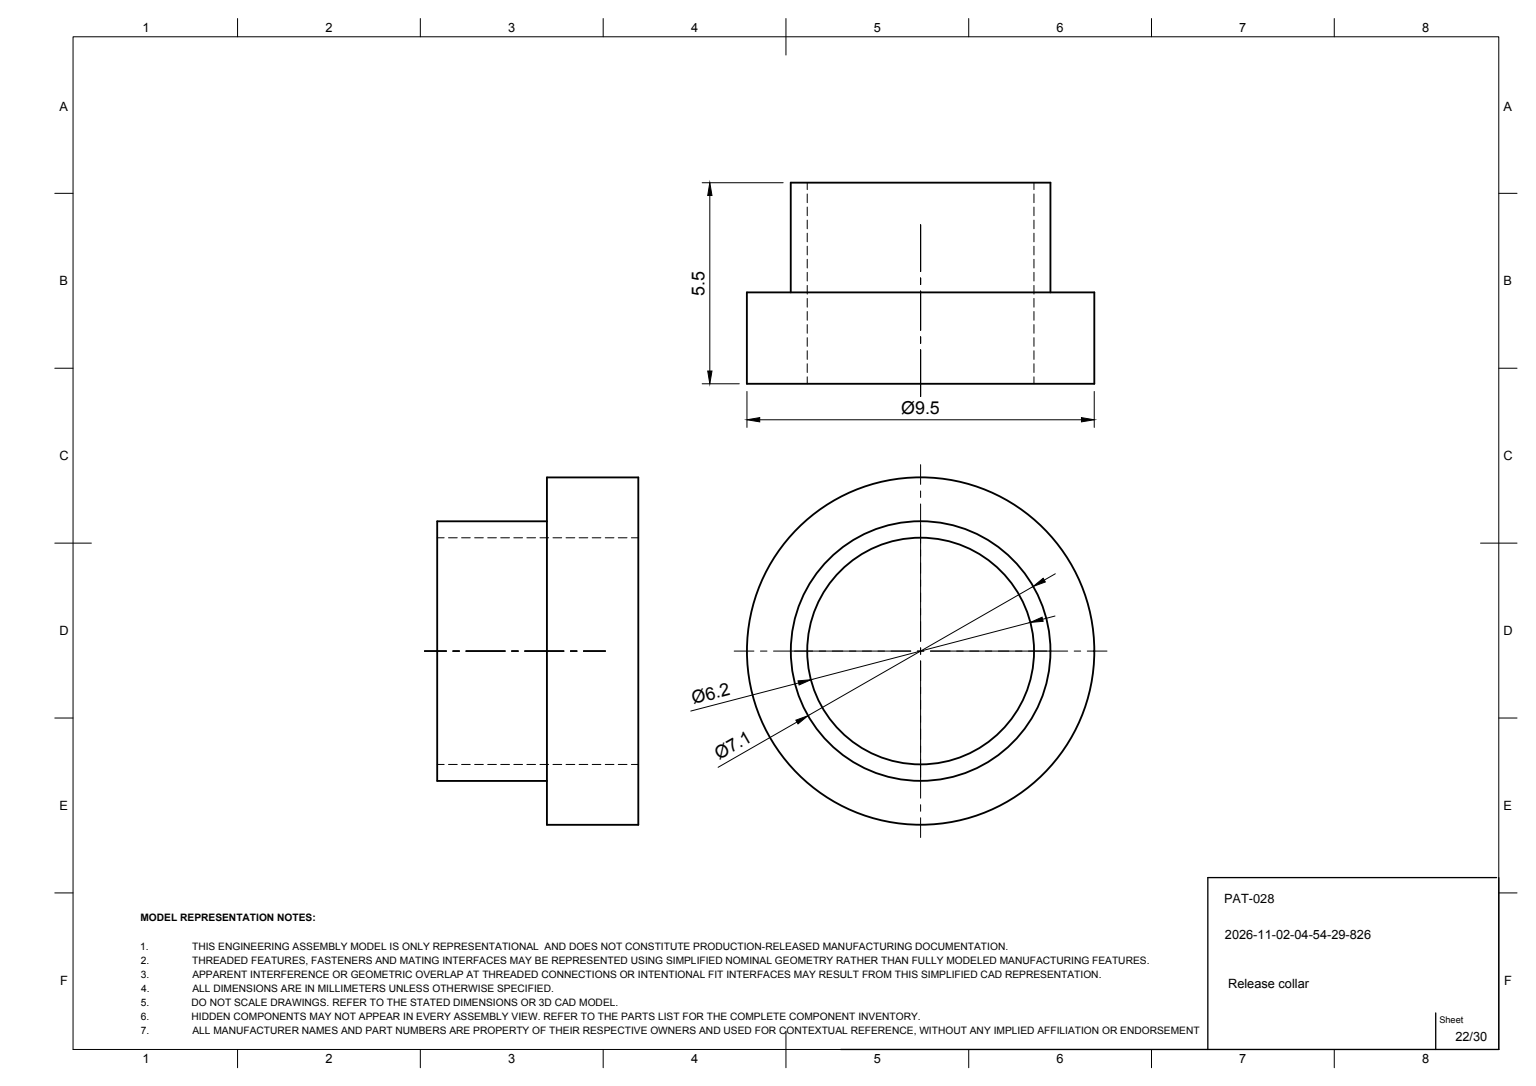
ISO-10303-21;
HEADER;
/* Generated by software containing ST-Developer
 * from STEP Tools, Inc. (www.steptools.com) 
 */

FILE_DESCRIPTION(
/* description */ ('Cylinder foot and clevis mount kit'),
/* implementation_level */ '2;1');

FILE_NAME(
/* name */ 'Release collar.step',
/* time_stamp */ '2026-10-27T20:10:43-07:00',
/* author */ (''),
/* organization */ (''),
/* preprocessor_version */ 'ST-DEVELOPER v20.2',
/* originating_system */ 'Autodesk Translation Framework v15.17.0.0',
/* authorisation */ '');

FILE_SCHEMA (('AUTOMOTIVE_DESIGN { 1 0 10303 214 3 1 1 }'));
ENDSEC;

DATA;
#10=MECHANICAL_DESIGN_GEOMETRIC_PRESENTATION_REPRESENTATION('',(#350),#9102);
#294=SHAPE_REPRESENTATION_RELATIONSHIP('SRR','None',#9242,#322);
#322=ADVANCED_BREP_SHAPE_REPRESENTATION('',(#377),#9085);
#350=STYLED_ITEM('',(#9474),#377);
#377=MANIFOLD_SOLID_BREP('Body1',#4937);
#463=FACE_BOUND('',#1266,.T.);
#464=FACE_BOUND('',#1269,.T.);
#465=FACE_BOUND('',#1272,.T.);
#628=PLANE('',#5624);
#629=PLANE('',#5629);
#630=PLANE('',#5633);
#888=FACE_OUTER_BOUND('',#1265,.T.);
#889=FACE_OUTER_BOUND('',#1267,.T.);
#890=FACE_OUTER_BOUND('',#1268,.T.);
#891=FACE_OUTER_BOUND('',#1270,.T.);
#892=FACE_OUTER_BOUND('',#1271,.T.);
#893=FACE_OUTER_BOUND('',#1273,.T.);
#1265=EDGE_LOOP('',(#4087));
#1266=EDGE_LOOP('',(#4088));
#1267=EDGE_LOOP('',(#4089,#4090,#4091,#4092));
#1268=EDGE_LOOP('',(#4093));
#1269=EDGE_LOOP('',(#4094));
#1270=EDGE_LOOP('',(#4095,#4096,#4097,#4098));
#1271=EDGE_LOOP('',(#4099));
#1272=EDGE_LOOP('',(#4100));
#1273=EDGE_LOOP('',(#4101,#4102,#4103,#4104));
#1644=LINE('',#8343,#1993);
#1645=LINE('',#8350,#1994);
#1646=LINE('',#8355,#1995);
#1993=VECTOR('',#6857,0.475);
#1994=VECTOR('',#6866,0.355);
#1995=VECTOR('',#6873,0.31);
#2246=CIRCLE('',#5625,0.475);
#2247=CIRCLE('',#5626,0.31);
#2248=CIRCLE('',#5628,0.475);
#2249=CIRCLE('',#5630,0.355);
#2250=CIRCLE('',#5632,0.355);
#2251=CIRCLE('',#5634,0.31);
#2572=VERTEX_POINT('',#8336);
#2573=VERTEX_POINT('',#8338);
#2574=VERTEX_POINT('',#8341);
#2575=VERTEX_POINT('',#8345);
#2576=VERTEX_POINT('',#8348);
#2577=VERTEX_POINT('',#8352);
#3098=EDGE_CURVE('',#2572,#2572,#2246,.T.);
#3099=EDGE_CURVE('',#2573,#2573,#2247,.T.);
#3100=EDGE_CURVE('',#2574,#2574,#2248,.T.);
#3101=EDGE_CURVE('',#2574,#2572,#1644,.T.);
#3102=EDGE_CURVE('',#2575,#2575,#2249,.T.);
#3103=EDGE_CURVE('',#2576,#2576,#2250,.T.);
#3104=EDGE_CURVE('',#2576,#2575,#1645,.T.);
#3105=EDGE_CURVE('',#2577,#2577,#2251,.T.);
#3106=EDGE_CURVE('',#2577,#2573,#1646,.T.);
#4087=ORIENTED_EDGE('',*,*,#3098,.F.);
#4088=ORIENTED_EDGE('',*,*,#3099,.T.);
#4089=ORIENTED_EDGE('',*,*,#3100,.F.);
#4090=ORIENTED_EDGE('',*,*,#3101,.T.);
#4091=ORIENTED_EDGE('',*,*,#3098,.T.);
#4092=ORIENTED_EDGE('',*,*,#3101,.F.);
#4093=ORIENTED_EDGE('',*,*,#3100,.T.);
#4094=ORIENTED_EDGE('',*,*,#3102,.F.);
#4095=ORIENTED_EDGE('',*,*,#3103,.F.);
#4096=ORIENTED_EDGE('',*,*,#3104,.T.);
#4097=ORIENTED_EDGE('',*,*,#3102,.T.);
#4098=ORIENTED_EDGE('',*,*,#3104,.F.);
#4099=ORIENTED_EDGE('',*,*,#3103,.T.);
#4100=ORIENTED_EDGE('',*,*,#3105,.F.);
#4101=ORIENTED_EDGE('',*,*,#3105,.T.);
#4102=ORIENTED_EDGE('',*,*,#3106,.T.);
#4103=ORIENTED_EDGE('',*,*,#3099,.F.);
#4104=ORIENTED_EDGE('',*,*,#3106,.F.);
#4587=CYLINDRICAL_SURFACE('',#5627,0.475);
#4588=CYLINDRICAL_SURFACE('',#5631,0.355);
#4589=CYLINDRICAL_SURFACE('',#5635,0.31);
#4811=ADVANCED_FACE('',(#888,#463),#628,.T.);
#4812=ADVANCED_FACE('',(#889),#4587,.T.);
#4813=ADVANCED_FACE('',(#890,#464),#629,.T.);
#4814=ADVANCED_FACE('',(#891),#4588,.T.);
#4815=ADVANCED_FACE('',(#892,#465),#630,.T.);
#4816=ADVANCED_FACE('',(#893),#4589,.F.);
#4937=CLOSED_SHELL('',(#4811,#4812,#4813,#4814,#4815,#4816));
#5623=AXIS2_PLACEMENT_3D('',#8334,#6845,#6846);
#5624=AXIS2_PLACEMENT_3D('',#8335,#6847,#6848);
#5625=AXIS2_PLACEMENT_3D('',#8337,#6849,#6850);
#5626=AXIS2_PLACEMENT_3D('',#8339,#6851,#6852);
#5627=AXIS2_PLACEMENT_3D('',#8340,#6853,#6854);
#5628=AXIS2_PLACEMENT_3D('',#8342,#6855,#6856);
#5629=AXIS2_PLACEMENT_3D('',#8344,#6858,#6859);
#5630=AXIS2_PLACEMENT_3D('',#8346,#6860,#6861);
#5631=AXIS2_PLACEMENT_3D('',#8347,#6862,#6863);
#5632=AXIS2_PLACEMENT_3D('',#8349,#6864,#6865);
#5633=AXIS2_PLACEMENT_3D('',#8351,#6867,#6868);
#5634=AXIS2_PLACEMENT_3D('',#8353,#6869,#6870);
#5635=AXIS2_PLACEMENT_3D('',#8354,#6871,#6872);
#6845=DIRECTION('axis',(0.,0.,1.));
#6846=DIRECTION('refdir',(1.,0.,0.));
#6847=DIRECTION('center_axis',(0.,1.,0.));
#6848=DIRECTION('ref_axis',(0.,0.,1.));
#6849=DIRECTION('center_axis',(0.,-1.,0.));
#6850=DIRECTION('ref_axis',(1.,0.,0.));
#6851=DIRECTION('center_axis',(0.,-1.,0.));
#6852=DIRECTION('ref_axis',(1.,0.,0.));
#6853=DIRECTION('center_axis',(0.,-1.,0.));
#6854=DIRECTION('ref_axis',(1.,0.,0.));
#6855=DIRECTION('center_axis',(0.,-1.,0.));
#6856=DIRECTION('ref_axis',(1.,0.,0.));
#6857=DIRECTION('',(0.,1.,0.));
#6858=DIRECTION('center_axis',(0.,-1.,0.));
#6859=DIRECTION('ref_axis',(0.,0.,-1.));
#6860=DIRECTION('center_axis',(0.,-1.,0.));
#6861=DIRECTION('ref_axis',(1.,0.,0.));
#6862=DIRECTION('center_axis',(0.,-1.,0.));
#6863=DIRECTION('ref_axis',(1.,0.,0.));
#6864=DIRECTION('center_axis',(0.,-1.,0.));
#6865=DIRECTION('ref_axis',(1.,0.,0.));
#6866=DIRECTION('',(0.,1.,0.));
#6867=DIRECTION('center_axis',(0.,-1.,0.));
#6868=DIRECTION('ref_axis',(0.,0.,-1.));
#6869=DIRECTION('center_axis',(0.,-1.,0.));
#6870=DIRECTION('ref_axis',(1.,0.,0.));
#6871=DIRECTION('center_axis',(0.,-1.,0.));
#6872=DIRECTION('ref_axis',(1.,0.,0.));
#6873=DIRECTION('',(0.,1.,0.));
#8334=CARTESIAN_POINT('',(0.,0.,0.));
#8335=CARTESIAN_POINT('Origin',(0.475,1.95,0.));
#8336=CARTESIAN_POINT('',(-0.475,1.95,-5.81707229594993E-17));
#8337=CARTESIAN_POINT('Origin',(0.,1.95,0.));
#8338=CARTESIAN_POINT('',(-0.31,1.95,-3.7964050773568E-17));
#8339=CARTESIAN_POINT('Origin',(0.,1.95,0.));
#8340=CARTESIAN_POINT('Origin',(0.,1.825,0.));
#8341=CARTESIAN_POINT('',(-0.475,1.7,-5.81707229594993E-17));
#8342=CARTESIAN_POINT('Origin',(0.,1.7,0.));
#8343=CARTESIAN_POINT('',(-0.475,1.825,-5.81707229594993E-17));
#8344=CARTESIAN_POINT('Origin',(0.355,1.7,0.));
#8345=CARTESIAN_POINT('',(-0.355,1.7,-4.3474961369731E-17));
#8346=CARTESIAN_POINT('Origin',(0.,1.7,0.));
#8347=CARTESIAN_POINT('Origin',(0.,1.55,0.));
#8348=CARTESIAN_POINT('',(-0.355,1.4,-4.3474961369731E-17));
#8349=CARTESIAN_POINT('Origin',(0.,1.4,0.));
#8350=CARTESIAN_POINT('',(-0.355,1.55,-4.3474961369731E-17));
#8351=CARTESIAN_POINT('Origin',(0.31,1.4,0.));
#8352=CARTESIAN_POINT('',(-0.31,1.4,-3.7964050773568E-17));
#8353=CARTESIAN_POINT('Origin',(0.,1.4,0.));
#8354=CARTESIAN_POINT('Origin',(0.,1.675,0.));
#8355=CARTESIAN_POINT('',(-0.31,1.675,-3.7964050773568E-17));
#9052=UNCERTAINTY_MEASURE_WITH_UNIT(LENGTH_MEASURE(0.001),#9103,
'DISTANCE_ACCURACY_VALUE',
'Maximum model space distance between geometric entities at asserted c
onnectivities');
#9069=UNCERTAINTY_MEASURE_WITH_UNIT(LENGTH_MEASURE(0.001),#9103,
'DISTANCE_ACCURACY_VALUE',
'Maximum model space distance between geometric entities at asserted c
onnectivities');
#9085=(
GEOMETRIC_REPRESENTATION_CONTEXT(3)
GLOBAL_UNCERTAINTY_ASSIGNED_CONTEXT((#9052))
GLOBAL_UNIT_ASSIGNED_CONTEXT((#9103,#9105,#9106))
REPRESENTATION_CONTEXT('','3D')
);
#9102=(
GEOMETRIC_REPRESENTATION_CONTEXT(3)
GLOBAL_UNCERTAINTY_ASSIGNED_CONTEXT((#9069))
GLOBAL_UNIT_ASSIGNED_CONTEXT((#9103,#9105,#9106))
REPRESENTATION_CONTEXT('','3D')
);
#9103=(
LENGTH_UNIT()
NAMED_UNIT(*)
SI_UNIT(.CENTI.,.METRE.)
);
#9105=(
NAMED_UNIT(*)
PLANE_ANGLE_UNIT()
SI_UNIT($,.RADIAN.)
);
#9106=(
NAMED_UNIT(*)
SI_UNIT($,.STERADIAN.)
SOLID_ANGLE_UNIT()
);
#9122=SHAPE_DEFINITION_REPRESENTATION(#9154,#9242);
#9154=PRODUCT_DEFINITION_SHAPE('',$,#9275);
#9242=SHAPE_REPRESENTATION('',(#5623),#9085);
#9259=PRODUCT_DEFINITION_CONTEXT('part definition',#9357,'design');
#9275=PRODUCT_DEFINITION('Release collar','Release collar',#9307,#9259);
#9307=PRODUCT_DEFINITION_FORMATION('',$,#9374);
#9357=APPLICATION_CONTEXT(
'Core Data for Automotive Mechanical Design Process');
#9358=PRODUCT_CONTEXT('part definition',#9357,'mechanical');
#9374=PRODUCT('Release collar','Release collar','Release collar',(#9358));
#9468=COLOUR_RGB('Off White',0.89,0.88,0.83);
#9469=FILL_AREA_STYLE_COLOUR('',#9468);
#9470=FILL_AREA_STYLE('',(#9469));
#9471=SURFACE_STYLE_FILL_AREA(#9470);
#9472=SURFACE_SIDE_STYLE('',(#9471));
#9473=SURFACE_STYLE_USAGE(.BOTH.,#9472);
#9474=PRESENTATION_STYLE_ASSIGNMENT((#9473));
ENDSEC;
END-ISO-10303-21;
